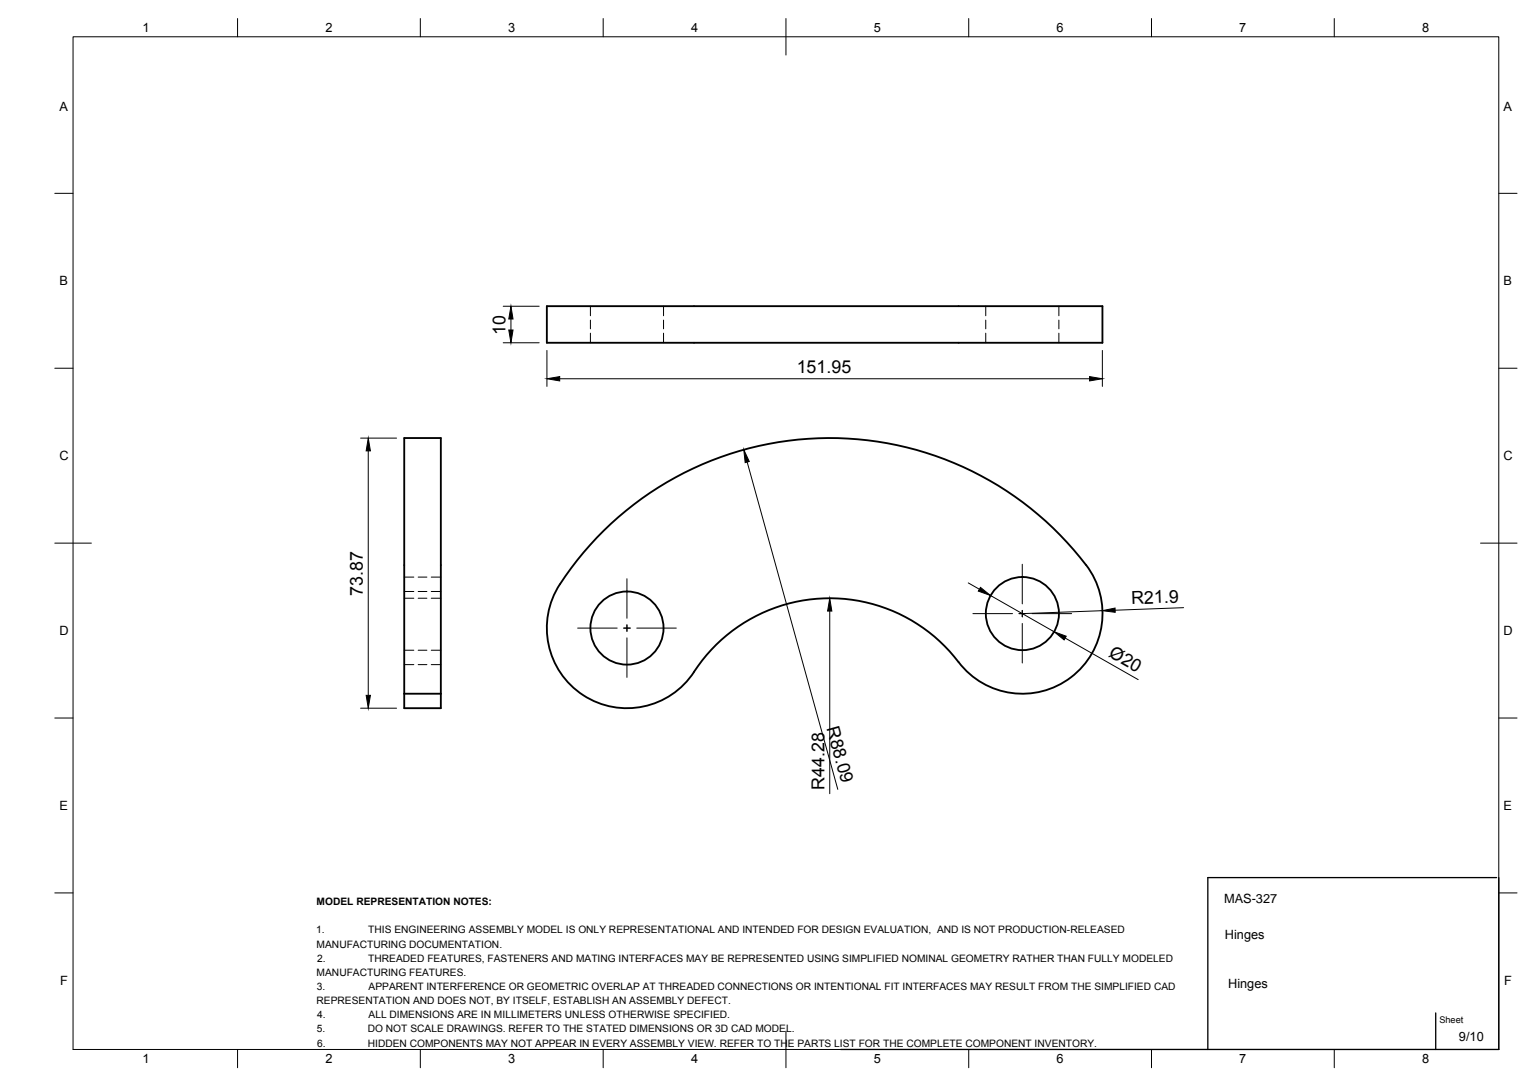
ISO-10303-21;
HEADER;
FILE_DESCRIPTION (('STEP AP214'),
    '1' );
FILE_NAME ('Hinges.step',
    '2026-10-06T22:16:42',
    ( '' ),
    ( '' ),
    'SwSTEP 2.0',
    'SolidWorks 2025',
    '' );
FILE_SCHEMA (( 'AUTOMOTIVE_DESIGN' ));
ENDSEC;

DATA;
#86=DIRECTION ( 'NONE',  ( 0.000000000000000000, 0.000000000000000000, 1.000000000000000000 ) ) ;
#206=AXIS2_PLACEMENT_3D ( 'NONE', #10122, #1740, #19817 ) ;
#240=DIRECTION ( 'NONE',  ( 0.000000000000000000, 0.000000000000000000, 1.000000000000000000 ) ) ;
#280=DIRECTION ( 'NONE',  ( -0.000000000000000000, -0.000000000000000000, -1.000000000000000000 ) ) ;
#386=DIRECTION ( 'NONE',  ( -1.000000000000000000, 0.000000000000000000, 0.000000000000000000 ) ) ;
#487=CARTESIAN_POINT ( 'NONE',  ( 147.5268905834513475, 193.0332408774651185, 14.00000000000001776 ) ) ;
#490=EDGE_CURVE ( 'NONE', #561, #602, #17397, .T. ) ;
#515=ORIENTED_EDGE ( 'NONE', *, *, #14295, .T. ) ;
#517=CARTESIAN_POINT ( 'NONE',  ( 159.4819454078502190, 211.3876867681337046, 14.00000000000001776 ) ) ;
#561=VERTEX_POINT ( 'NONE', #8931 ) ;
#598=CARTESIAN_POINT ( 'NONE',  ( 147.5268905834513475, 193.0332408774651185, 14.00000000000001776 ) ) ;
#602=VERTEX_POINT ( 'NONE', #3063 ) ;
#624=AXIS2_PLACEMENT_3D ( 'NONE', #1762, #13223, #18408 ) ;
#683=ORIENTED_EDGE ( 'NONE', *, *, #21000, .F. ) ;
#816=ORIENTED_EDGE ( 'NONE', *, *, #1747, .T. ) ;
#867=CYLINDRICAL_SURFACE ( 'NONE', #16262, 88.09373137032866907 ) ;
#906=CARTESIAN_POINT ( 'NONE',  ( 138.2149183826930425, 102.3264679885537305, 14.00000000000001776 ) ) ;
#911=CIRCLE ( 'NONE', #16036, 88.09373137032866907 ) ;
#917=CIRCLE ( 'NONE', #14285, 21.90454335994854063 ) ;
#947=CIRCLE ( 'NONE', #8357, 10.00000000000000888 ) ;
#963=SHAPE_REPRESENTATION_RELATIONSHIP ( 'NONE' , 'NONE' ,  #3970, #16628 ) ;
#966=ADVANCED_FACE ( 'NONE', ( #3402 ), #18495, .T. ) ;
#1001=EDGE_LOOP ( 'NONE', ( #7950, #11263, #15363, #5851 ) ) ;
#1043=FACE_OUTER_BOUND ( 'NONE', #2864, .T. ) ;
#1045=( LENGTH_UNIT ( ) NAMED_UNIT ( * ) SI_UNIT ( .MILLI., .METRE. ) );
#1216=ORIENTED_EDGE ( 'NONE', *, *, #20304, .F. ) ;
#1369=( NAMED_UNIT ( * ) PLANE_ANGLE_UNIT ( ) SI_UNIT ( $, .RADIAN. ) );
#1376=AXIS2_PLACEMENT_3D ( 'NONE', #4360, #21349, #17699 ) ;
#1501=PRODUCT ( 'Hinges', 'Hinges', '', ( #2695 ) ) ;
#1740=DIRECTION ( 'NONE',  ( 0.000000000000000000, 0.000000000000000000, 1.000000000000000000 ) ) ;
#1747=EDGE_CURVE ( 'NONE', #4207, #19742, #20682, .T. ) ;
#1762=CARTESIAN_POINT ( 'NONE',  ( 151.4773229304660731, 84.89323405393692212, 14.00000000000001776 ) ) ;
#1767=ORIENTED_EDGE ( 'NONE', *, *, #7862, .T. ) ;
#1776=( GEOMETRIC_REPRESENTATION_CONTEXT ( 3 ) GLOBAL_UNCERTAINTY_ASSIGNED_CONTEXT ( ( #14131 ) ) GLOBAL_UNIT_ASSIGNED_CONTEXT ( ( #2724, #2506, #19371 ) ) REPRESENTATION_CONTEXT ( 'NONE', 'WORKASPACE' ) );
#1809=CARTESIAN_POINT ( 'NONE',  ( 129.5727795705175822, 84.89323405393692212, 14.00000000000001776 ) ) ;
#1834=AXIS2_PLACEMENT_3D ( 'NONE', #598, #280, #19122 ) ;
#1849=CARTESIAN_POINT ( 'NONE',  ( 137.5268905834513191, 193.0332408774651185, 14.00000000000001776 ) ) ;
#1928=CARTESIAN_POINT ( 'NONE',  ( 129.5727795705175822, 84.89323405393692212, 4.000000000000021316 ) ) ;
#2018=EDGE_LOOP ( 'NONE', ( #1767, #3911, #17935, #2040 ) ) ;
#2040=ORIENTED_EDGE ( 'NONE', *, *, #6906, .T. ) ;
#2069=EDGE_CURVE ( 'NONE', #4207, #6019, #20285, .T. ) ;
#2144=CARTESIAN_POINT ( 'NONE',  ( 147.5268905834513475, 193.0332408774651185, 4.000000000000021316 ) ) ;
#2330=ORIENTED_EDGE ( 'NONE', *, *, #21000, .T. ) ;
#2368=CARTESIAN_POINT ( 'NONE',  ( 164.7397274782390184, 67.46000011932014218, 4.000000000000021316 ) ) ;
#2403=CARTESIAN_POINT ( 'NONE',  ( 0.000000000000000000, 0.000000000000000000, 0.000000000000000000 ) ) ;
#2440=ORIENTED_EDGE ( 'NONE', *, *, #14295, .F. ) ;
#2445=CARTESIAN_POINT ( 'NONE',  ( 135.5718357590524192, 174.6787949867965324, 4.000000000000021316 ) ) ;
#2506=( NAMED_UNIT ( * ) PLANE_ANGLE_UNIT ( ) SI_UNIT ( $, .RADIAN. ) );
#2688=CARTESIAN_POINT ( 'NONE',  ( 151.4773229304660731, 84.89323405393692212, 14.00000000000001776 ) ) ;
#2695=PRODUCT_CONTEXT ( 'NONE', #5614, 'mechanical' ) ;
#2724=( LENGTH_UNIT ( ) NAMED_UNIT ( * ) SI_UNIT ( .MILLI., .METRE. ) );
#2734=DIRECTION ( 'NONE',  ( -0.000000000000000000, -0.000000000000000000, -1.000000000000000000 ) ) ;
#2752=CARTESIAN_POINT ( 'NONE',  ( 151.4773229304660731, 84.89323405393692212, 14.00000000000001776 ) ) ;
#2786=AXIS2_PLACEMENT_3D ( 'NONE', #13218, #4841, #6619 ) ;
#2842=ORIENTED_EDGE ( 'NONE', *, *, #14486, .F. ) ;
#2864=EDGE_LOOP ( 'NONE', ( #515, #9206, #2842, #9559 ) ) ;
#2893=AXIS2_PLACEMENT_3D ( 'NONE', #7958, #11580, #15332 ) ;
#2901=VECTOR ( 'NONE', #20014, 1000.000000000000000 ) ;
#2935=LINE ( 'NONE', #21135, #17207 ) ;
#2946=DIRECTION ( 'NONE',  ( 1.000000000000000000, 0.000000000000000000, 0.000000000000000000 ) ) ;
#2953=ORIENTED_EDGE ( 'NONE', *, *, #7751, .T. ) ;
#3063=CARTESIAN_POINT ( 'NONE',  ( 141.4773229304660447, 84.89323405393692212, 4.000000000000021316 ) ) ;
#3069=CARTESIAN_POINT ( 'NONE',  ( 157.5268905834513475, 193.0332408774651185, 4.000000000000021316 ) ) ;
#3087=AXIS2_PLACEMENT_3D ( 'NONE', #5335, #10087, #8763 ) ;
#3283=CARTESIAN_POINT ( 'NONE',  ( 147.5268905834513475, 193.0332408774651185, 14.00000000000001776 ) ) ;
#3290=EDGE_CURVE ( 'NONE', #19742, #18253, #917, .T. ) ;
#3292=CARTESIAN_POINT ( 'NONE',  ( 138.2149183826930425, 102.3264679885537305, 4.000000000000021316 ) ) ;
#3361=UNCERTAINTY_MEASURE_WITH_UNIT (LENGTH_MEASURE( 1.000000000000000082E-05 ), #1045, 'distance_accuracy_value', 'NONE');
#3402=FACE_OUTER_BOUND ( 'NONE', #5526, .T. ) ;
#3453=CARTESIAN_POINT ( 'NONE',  ( 147.5268905834513475, 193.0332408774651185, 4.000000000000021316 ) ) ;
#3558=ORIENTED_EDGE ( 'NONE', *, *, #3290, .F. ) ;
#3605=FACE_BOUND ( 'NONE', #4278, .T. ) ;
#3678=ADVANCED_FACE ( 'NONE', ( #18042, #6479, #16173 ), #7816, .F. ) ;
#3802=CIRCLE ( 'NONE', #18591, 10.00000000000000888 ) ;
#3803=FACE_OUTER_BOUND ( 'NONE', #16547, .T. ) ;
#3855=EDGE_CURVE ( 'NONE', #8015, #10293, #8796, .T. ) ;
#3911=ORIENTED_EDGE ( 'NONE', *, *, #1747, .F. ) ;
#3934=DIRECTION ( 'NONE',  ( -0.000000000000000000, -0.000000000000000000, -1.000000000000000000 ) ) ;
#3947=EDGE_CURVE ( 'NONE', #16997, #8015, #3802, .T. ) ;
#3970=SHAPE_REPRESENTATION ( 'Hinges', ( #12657 ), #1776 ) ;
#3979=DIRECTION ( 'NONE',  ( 1.000000000000000000, 0.000000000000000000, 0.000000000000000000 ) ) ;
#4168=CARTESIAN_POINT ( 'NONE',  ( 151.4773229304660731, 84.89323405393692212, 4.000000000000021316 ) ) ;
#4173=EDGE_CURVE ( 'NONE', #18391, #12691, #19038, .T. ) ;
#4207=VERTEX_POINT ( 'NONE', #517 ) ;
#4278=EDGE_LOOP ( 'NONE', ( #15239, #11300 ) ) ;
#4339=CARTESIAN_POINT ( 'NONE',  ( 137.5268905834513191, 193.0332408774651185, 4.000000000000021316 ) ) ;
#4360=CARTESIAN_POINT ( 'NONE',  ( 147.5268905834513475, 193.0332408774651185, 14.00000000000001776 ) ) ;
#4487=FACE_OUTER_BOUND ( 'NONE', #2018, .T. ) ;
#4579=ORIENTED_EDGE ( 'NONE', *, *, #490, .T. ) ;
#4603=VERTEX_POINT ( 'NONE', #1928 ) ;
#4652=PRODUCT_DEFINITION_CONTEXT ( 'detailed design', #18727, 'design' ) ;
#4765=EDGE_LOOP ( 'NONE', ( #17772, #14554 ) ) ;
#4777=CARTESIAN_POINT ( 'NONE',  ( 164.7397274782390184, 67.46000011932014218, 14.00000000000001776 ) ) ;
#4841=DIRECTION ( 'NONE',  ( 0.000000000000000000, 0.000000000000000000, 1.000000000000000000 ) ) ;
#4901=EDGE_CURVE ( 'NONE', #13154, #4207, #12224, .T. ) ;
#4928=DIRECTION ( 'NONE',  ( 0.000000000000000000, 0.000000000000000000, 1.000000000000000000 ) ) ;
#4974=ORIENTED_EDGE ( 'NONE', *, *, #10822, .F. ) ;
#5039=FACE_OUTER_BOUND ( 'NONE', #10933, .T. ) ;
#5114=DIRECTION ( 'NONE',  ( -1.000000000000000000, 0.000000000000000000, 0.000000000000000000 ) ) ;
#5268=CIRCLE ( 'NONE', #6317, 10.00000000000000888 ) ;
#5335=CARTESIAN_POINT ( 'NONE',  ( 111.4021762516569964, 137.5714195593754710, 14.00000000000001776 ) ) ;
#5446=ORIENTED_EDGE ( 'NONE', *, *, #9283, .T. ) ;
#5526=EDGE_LOOP ( 'NONE', ( #7904, #7670, #21323, #21268 ) ) ;
#5567=CARTESIAN_POINT ( 'NONE',  ( 159.4819454078502190, 211.3876867681337046, 14.00000000000001776 ) ) ;
#5614=APPLICATION_CONTEXT ( 'automotive_design' ) ;
#5615=( GEOMETRIC_REPRESENTATION_CONTEXT ( 3 ) GLOBAL_UNCERTAINTY_ASSIGNED_CONTEXT ( ( #3361 ) ) GLOBAL_UNIT_ASSIGNED_CONTEXT ( ( #1045, #1369, #18113 ) ) REPRESENTATION_CONTEXT ( 'NONE', 'WORKASPACE' ) );
#5673=FACE_OUTER_BOUND ( 'NONE', #15781, .T. ) ;
#5779=CIRCLE ( 'NONE', #7222, 10.00000000000000888 ) ;
#5832=DIRECTION ( 'NONE',  ( -0.000000000000000000, -0.000000000000000000, -1.000000000000000000 ) ) ;
#5851=ORIENTED_EDGE ( 'NONE', *, *, #490, .F. ) ;
#5946=DIRECTION ( 'NONE',  ( -1.000000000000000000, 0.000000000000000000, 0.000000000000000000 ) ) ;
#6016=ORIENTED_EDGE ( 'NONE', *, *, #10822, .T. ) ;
#6019=VERTEX_POINT ( 'NONE', #21122 ) ;
#6046=PRODUCT_DEFINITION_SHAPE ( 'NONE', 'NONE',  #14706 ) ;
#6105=EDGE_CURVE ( 'NONE', #20206, #561, #8184, .T. ) ;
#6201=CARTESIAN_POINT ( 'NONE',  ( 147.5268905834513475, 193.0332408774651185, 4.000000000000021316 ) ) ;
#6257=VECTOR ( 'NONE', #7033, 1000.000000000000000 ) ;
#6296=CIRCLE ( 'NONE', #14048, 21.90454335994854063 ) ;
#6317=AXIS2_PLACEMENT_3D ( 'NONE', #2688, #17781, #7779 ) ;
#6329=SURFACE_SIDE_STYLE ('',( #14808 ) ) ;
#6365=CARTESIAN_POINT ( 'NONE',  ( 111.4021762516569964, 137.5714195593754710, 4.000000000000021316 ) ) ;
#6367=CARTESIAN_POINT ( 'NONE',  ( 131.4397495910615135, 111.2323268066561894, 4.000000000000021316 ) ) ;
#6390=ADVANCED_FACE ( 'NONE', ( #3605, #5039, #17031 ), #6811, .T. ) ;
#6439=CARTESIAN_POINT ( 'NONE',  ( 147.5268905834513475, 193.0332408774651185, 14.00000000000001776 ) ) ;
#6479=FACE_BOUND ( 'NONE', #21784, .T. ) ;
#6489=DIRECTION ( 'NONE',  ( 1.000000000000000000, 0.000000000000000000, 0.000000000000000000 ) ) ;
#6619=DIRECTION ( 'NONE',  ( 1.000000000000000000, 0.000000000000000000, 0.000000000000000000 ) ) ;
#6630=ORIENTED_EDGE ( 'NONE', *, *, #14584, .F. ) ;
#6719=DIRECTION ( 'NONE',  ( -1.000000000000000000, 0.000000000000000000, 0.000000000000000000 ) ) ;
#6811=PLANE ( 'NONE',  #18735 ) ;
#6883=CYLINDRICAL_SURFACE ( 'NONE', #18176, 21.90454335994848734 ) ;
#6900=CYLINDRICAL_SURFACE ( 'NONE', #19935, 21.90454335994854063 ) ;
#6906=EDGE_CURVE ( 'NONE', #13154, #10374, #20438, .T. ) ;
#6958=AXIS2_PLACEMENT_3D ( 'NONE', #7777, #21221, #9647 ) ;
#7033=DIRECTION ( 'NONE',  ( -0.000000000000000000, -0.000000000000000000, -1.000000000000000000 ) ) ;
#7050=DIRECTION ( 'NONE',  ( 0.000000000000000000, 0.000000000000000000, 1.000000000000000000 ) ) ;
#7108=CARTESIAN_POINT ( 'NONE',  ( 147.5268905834513475, 193.0332408774651185, 14.00000000000001776 ) ) ;
#7162=CARTESIAN_POINT ( 'NONE',  ( 147.5268905834513475, 193.0332408774651185, 14.00000000000001776 ) ) ;
#7222=AXIS2_PLACEMENT_3D ( 'NONE', #4168, #9140, #10897 ) ;
#7225=DIRECTION ( 'NONE',  ( -0.000000000000000000, -0.000000000000000000, -1.000000000000000000 ) ) ;
#7363=EDGE_CURVE ( 'NONE', #13378, #13154, #7385, .T. ) ;
#7369=CIRCLE ( 'NONE', #1376, 10.00000000000000888 ) ;
#7385=CIRCLE ( 'NONE', #2786, 21.90454335994848734 ) ;
#7398=COLOUR_RGB ( '', 0.09019608, 0.27058824, 0.51372549) ;
#7494=EDGE_CURVE ( 'NONE', #20206, #19334, #17273, .T. ) ;
#7511=LINE ( 'NONE', #14210, #17134 ) ;
#7616=AXIS2_PLACEMENT_3D ( 'NONE', #2144, #8877, #15584 ) ;
#7622=CYLINDRICAL_SURFACE ( 'NONE', #7907, 10.00000000000000888 ) ;
#7670=ORIENTED_EDGE ( 'NONE', *, *, #9283, .F. ) ;
#7682=SHAPE_DEFINITION_REPRESENTATION ( #6046, #3970 ) ;
#7750=ORIENTED_EDGE ( 'NONE', *, *, #6906, .F. ) ;
#7751=EDGE_CURVE ( 'NONE', #13378, #4603, #16490, .T. ) ;
#7772=ORIENTED_EDGE ( 'NONE', *, *, #20824, .T. ) ;
#7777=CARTESIAN_POINT ( 'NONE',  ( 111.4021762516569964, 137.5714195593754710, 14.00000000000001776 ) ) ;
#7779=DIRECTION ( 'NONE',  ( 1.000000000000000000, 0.000000000000000000, 0.000000000000000000 ) ) ;
#7816=PLANE ( 'NONE',  #10148 ) ;
#7862=EDGE_CURVE ( 'NONE', #10374, #19742, #911, .T. ) ;
#7877=EDGE_CURVE ( 'NONE', #20239, #10293, #9724, .T. ) ;
#7891=EDGE_CURVE ( 'NONE', #4603, #10374, #15355, .T. ) ;
#7904=ORIENTED_EDGE ( 'NONE', *, *, #7751, .F. ) ;
#7907=AXIS2_PLACEMENT_3D ( 'NONE', #12782, #15866, #5946 ) ;
#7950=ORIENTED_EDGE ( 'NONE', *, *, #21656, .T. ) ;
#7957=ORIENTED_EDGE ( 'NONE', *, *, #2069, .T. ) ;
#7958=CARTESIAN_POINT ( 'NONE',  ( 151.4773229304660731, 84.89323405393692212, 4.000000000000021316 ) ) ;
#7988=ORIENTED_EDGE ( 'NONE', *, *, #14486, .T. ) ;
#8015=VERTEX_POINT ( 'NONE', #12411 ) ;
#8184=CIRCLE ( 'NONE', #8539, 10.00000000000000888 ) ;
#8322=CARTESIAN_POINT ( 'NONE',  ( 164.7397274782390184, 67.46000011932014218, 14.00000000000001776 ) ) ;
#8339=DIRECTION ( 'NONE',  ( -0.000000000000000000, -0.000000000000000000, -1.000000000000000000 ) ) ;
#8357=AXIS2_PLACEMENT_3D ( 'NONE', #12124, #15762, #3979 ) ;
#8363=CARTESIAN_POINT ( 'NONE',  ( 151.4773229304660731, 84.89323405393692212, 14.00000000000001776 ) ) ;
#8422=CARTESIAN_POINT ( 'NONE',  ( 157.5268905834513475, 193.0332408774651185, 14.00000000000001776 ) ) ;
#8474=CARTESIAN_POINT ( 'NONE',  ( 129.5727795705175822, 84.89323405393692212, 14.00000000000001776 ) ) ;
#8475=CLOSED_SHELL ( 'NONE', ( #9761, #18925, #8585, #13380, #6390, #3678, #966, #17842, #16477, #10699, #12632, #10454 ) ) ;
#8539=AXIS2_PLACEMENT_3D ( 'NONE', #11096, #13079, #17808 ) ;
#8565=EDGE_CURVE ( 'NONE', #18253, #13487, #18870, .T. ) ;
#8585=ADVANCED_FACE ( 'NONE', ( #3803 ), #6900, .T. ) ;
#8596=FACE_OUTER_BOUND ( 'NONE', #20913, .T. ) ;
#8763=DIRECTION ( 'NONE',  ( 1.000000000000000000, 0.000000000000000000, 0.000000000000000000 ) ) ;
#8773=CYLINDRICAL_SURFACE ( 'NONE', #1834, 21.90454335994854063 ) ;
#8796=LINE ( 'NONE', #1849, #6257 ) ;
#8877=DIRECTION ( 'NONE',  ( 0.000000000000000000, 0.000000000000000000, 1.000000000000000000 ) ) ;
#8931=CARTESIAN_POINT ( 'NONE',  ( 141.4773229304660447, 84.89323405393692212, 14.00000000000001776 ) ) ;
#8933=EDGE_LOOP ( 'NONE', ( #11196, #15122, #816, #15559 ) ) ;
#8990=DIRECTION ( 'NONE',  ( -0.000000000000000000, -0.000000000000000000, -1.000000000000000000 ) ) ;
#9103=EDGE_LOOP ( 'NONE', ( #19441, #11957, #4579, #4974 ) ) ;
#9140=DIRECTION ( 'NONE',  ( 0.000000000000000000, 0.000000000000000000, 1.000000000000000000 ) ) ;
#9206=ORIENTED_EDGE ( 'NONE', *, *, #4173, .F. ) ;
#9283=EDGE_CURVE ( 'NONE', #18391, #13378, #20702, .T. ) ;
#9312=DIRECTION ( 'NONE',  ( 1.000000000000000000, 0.000000000000000000, 0.000000000000000000 ) ) ;
#9368=VECTOR ( 'NONE', #14738, 1000.000000000000000 ) ;
#9396=CIRCLE ( 'NONE', #12198, 44.28464465043163756 ) ;
#9422=DIRECTION ( 'NONE',  ( 1.000000000000000000, 0.000000000000000000, 0.000000000000000000 ) ) ;
#9492=FACE_OUTER_BOUND ( 'NONE', #1001, .T. ) ;
#9559=ORIENTED_EDGE ( 'NONE', *, *, #14093, .T. ) ;
#9647=DIRECTION ( 'NONE',  ( -1.000000000000000000, 0.000000000000000000, 0.000000000000000000 ) ) ;
#9687=CARTESIAN_POINT ( 'NONE',  ( 151.4773229304660731, 84.89323405393692212, 4.000000000000021316 ) ) ;
#9697=CARTESIAN_POINT ( 'NONE',  ( 161.4773229304660731, 84.89323405393692212, 14.00000000000001776 ) ) ;
#9724=CIRCLE ( 'NONE', #206, 10.00000000000000888 ) ;
#9761=ADVANCED_FACE ( 'NONE', ( #8596 ), #20280, .F. ) ;
#9995=CARTESIAN_POINT ( 'NONE',  ( 135.5718357590524192, 174.6787949867965324, 14.00000000000001776 ) ) ;
#10087=DIRECTION ( 'NONE',  ( 0.000000000000000000, 0.000000000000000000, 1.000000000000000000 ) ) ;
#10122=CARTESIAN_POINT ( 'NONE',  ( 147.5268905834513475, 193.0332408774651185, 4.000000000000021316 ) ) ;
#10148=AXIS2_PLACEMENT_3D ( 'NONE', #6367, #14521, #21261 ) ;
#10218=PRODUCT_DEFINITION_FORMATION_WITH_SPECIFIED_SOURCE ( 'ANY', '', #1501, .NOT_KNOWN. ) ;
#10286=ORIENTED_EDGE ( 'NONE', *, *, #7877, .F. ) ;
#10293=VERTEX_POINT ( 'NONE', #4339 ) ;
#10374=VERTEX_POINT ( 'NONE', #2368 ) ;
#10454=ADVANCED_FACE ( 'NONE', ( #5673 ), #19130, .F. ) ;
#10536=ORIENTED_EDGE ( 'NONE', *, *, #15749, .F. ) ;
#10561=STYLED_ITEM ( 'NONE', ( #13055 ), #21708 ) ;
#10584=DIRECTION ( 'NONE',  ( -0.000000000000000000, -0.000000000000000000, -1.000000000000000000 ) ) ;
#10640=FACE_OUTER_BOUND ( 'NONE', #8933, .T. ) ;
#10680=DIRECTION ( 'NONE',  ( -1.000000000000000000, 0.000000000000000000, 0.000000000000000000 ) ) ;
#10699=ADVANCED_FACE ( 'NONE', ( #1043 ), #14699, .F. ) ;
#10822=EDGE_CURVE ( 'NONE', #19334, #602, #947, .T. ) ;
#10862=CARTESIAN_POINT ( 'NONE',  ( 111.4021762516569964, 137.5714195593754710, 4.000000000000021316 ) ) ;
#10897=DIRECTION ( 'NONE',  ( 1.000000000000000000, 0.000000000000000000, 0.000000000000000000 ) ) ;
#10933=EDGE_LOOP ( 'NONE', ( #5446, #16391, #17909, #7957, #18415, #7988 ) ) ;
#11096=CARTESIAN_POINT ( 'NONE',  ( 151.4773229304660731, 84.89323405393692212, 14.00000000000001776 ) ) ;
#11109=CARTESIAN_POINT ( 'NONE',  ( 111.4021762516569964, 137.5714195593754710, 14.00000000000001776 ) ) ;
#11196=ORIENTED_EDGE ( 'NONE', *, *, #20824, .F. ) ;
#11217=ORIENTED_EDGE ( 'NONE', *, *, #14093, .F. ) ;
#11233=EDGE_CURVE ( 'NONE', #16997, #20239, #7511, .T. ) ;
#11263=ORIENTED_EDGE ( 'NONE', *, *, #7494, .T. ) ;
#11283=FILL_AREA_STYLE_COLOUR ( '', #7398 ) ;
#11300=ORIENTED_EDGE ( 'NONE', *, *, #6105, .F. ) ;
#11310=CARTESIAN_POINT ( 'NONE',  ( 159.4819454078502190, 211.3876867681337046, 4.000000000000021316 ) ) ;
#11501=DIRECTION ( 'NONE',  ( -1.000000000000000000, 0.000000000000000000, 0.000000000000000000 ) ) ;
#11580=DIRECTION ( 'NONE',  ( 0.000000000000000000, 0.000000000000000000, 1.000000000000000000 ) ) ;
#11639=DIRECTION ( 'NONE',  ( 1.000000000000000000, 0.000000000000000000, -0.000000000000000000 ) ) ;
#11780=CARTESIAN_POINT ( 'NONE',  ( 161.4773229304660731, 84.89323405393692212, 14.00000000000001776 ) ) ;
#11856=AXIS2_PLACEMENT_3D ( 'NONE', #7162, #17275, #10680 ) ;
#11859=CIRCLE ( 'NONE', #19959, 44.28464465043163756 ) ;
#11957=ORIENTED_EDGE ( 'NONE', *, *, #6105, .T. ) ;
#11970=CARTESIAN_POINT ( 'NONE',  ( 131.4397495910615135, 111.2323268066561894, 14.00000000000001776 ) ) ;
#12124=CARTESIAN_POINT ( 'NONE',  ( 151.4773229304660731, 84.89323405393692212, 4.000000000000021316 ) ) ;
#12194=AXIS2_PLACEMENT_3D ( 'NONE', #2752, #12676, #21280 ) ;
#12198=AXIS2_PLACEMENT_3D ( 'NONE', #10862, #8990, #9312 ) ;
#12224=CIRCLE ( 'NONE', #3087, 88.09373137032866907 ) ;
#12289=DIRECTION ( 'NONE',  ( -0.000000000000000000, -0.000000000000000000, -1.000000000000000000 ) ) ;
#12411=CARTESIAN_POINT ( 'NONE',  ( 137.5268905834513191, 193.0332408774651185, 14.00000000000001776 ) ) ;
#12528=AXIS2_PLACEMENT_3D ( 'NONE', #9687, #18490, #21806 ) ;
#12552=CARTESIAN_POINT ( 'NONE',  ( 141.4773229304660447, 84.89323405393692212, 14.00000000000001776 ) ) ;
#12632=ADVANCED_FACE ( 'NONE', ( #15317 ), #21720, .F. ) ;
#12657=AXIS2_PLACEMENT_3D ( 'NONE', #2403, #7050, #17169 ) ;
#12676=DIRECTION ( 'NONE',  ( 0.000000000000000000, 0.000000000000000000, 1.000000000000000000 ) ) ;
#12691=VERTEX_POINT ( 'NONE', #3292 ) ;
#12782=CARTESIAN_POINT ( 'NONE',  ( 151.4773229304660731, 84.89323405393692212, 14.00000000000001776 ) ) ;
#12802=ORIENTED_EDGE ( 'NONE', *, *, #19592, .T. ) ;
#12986=DIRECTION ( 'NONE',  ( -1.000000000000000000, 0.000000000000000000, 0.000000000000000000 ) ) ;
#13055=PRESENTATION_STYLE_ASSIGNMENT (( #19448 ) ) ;
#13079=DIRECTION ( 'NONE',  ( 0.000000000000000000, 0.000000000000000000, 1.000000000000000000 ) ) ;
#13154=VERTEX_POINT ( 'NONE', #4777 ) ;
#13218=CARTESIAN_POINT ( 'NONE',  ( 151.4773229304660731, 84.89323405393692212, 14.00000000000001776 ) ) ;
#13223=DIRECTION ( 'NONE',  ( -0.000000000000000000, -0.000000000000000000, -1.000000000000000000 ) ) ;
#13378=VERTEX_POINT ( 'NONE', #1809 ) ;
#13380=ADVANCED_FACE ( 'NONE', ( #17000 ), #6883, .T. ) ;
#13480=ORIENTED_EDGE ( 'NONE', *, *, #7891, .F. ) ;
#13487=VERTEX_POINT ( 'NONE', #2445 ) ;
#13489=DIRECTION ( 'NONE',  ( -0.000000000000000000, -0.000000000000000000, -1.000000000000000000 ) ) ;
#13527=DIRECTION ( 'NONE',  ( 1.000000000000000000, 0.000000000000000000, 0.000000000000000000 ) ) ;
#13813=DIRECTION ( 'NONE',  ( 0.000000000000000000, 0.000000000000000000, 1.000000000000000000 ) ) ;
#13910=VECTOR ( 'NONE', #12289, 1000.000000000000000 ) ;
#13941=VECTOR ( 'NONE', #8339, 1000.000000000000000 ) ;
#13995=VECTOR ( 'NONE', #3934, 1000.000000000000000 ) ;
#14048=AXIS2_PLACEMENT_3D ( 'NONE', #14748, #18162, #6489 ) ;
#14093=EDGE_CURVE ( 'NONE', #14386, #13487, #20136, .T. ) ;
#14131=UNCERTAINTY_MEASURE_WITH_UNIT (LENGTH_MEASURE( 1.000000000000000082E-05 ), #2724, 'distance_accuracy_value', 'NONE');
#14178=EDGE_LOOP ( 'NONE', ( #6630, #2440, #16753, #3558, #17616, #13480 ) ) ;
#14210=CARTESIAN_POINT ( 'NONE',  ( 157.5268905834513475, 193.0332408774651185, 14.00000000000001776 ) ) ;
#14285=AXIS2_PLACEMENT_3D ( 'NONE', #6201, #17988, #21102 ) ;
#14295=EDGE_CURVE ( 'NONE', #13487, #12691, #9396, .T. ) ;
#14386=VERTEX_POINT ( 'NONE', #21657 ) ;
#14413=MECHANICAL_DESIGN_GEOMETRIC_PRESENTATION_REPRESENTATION('',(#10561),#5615);
#14486=EDGE_CURVE ( 'NONE', #14386, #18391, #11859, .T. ) ;
#14521=DIRECTION ( 'NONE',  ( 0.000000000000000000, 0.000000000000000000, 1.000000000000000000 ) ) ;
#14554=ORIENTED_EDGE ( 'NONE', *, *, #7877, .T. ) ;
#14556=ORIENTED_EDGE ( 'NONE', *, *, #3947, .F. ) ;
#14584=EDGE_CURVE ( 'NONE', #12691, #4603, #18744, .T. ) ;
#14692=DIRECTION ( 'NONE',  ( -0.000000000000000000, -0.000000000000000000, -1.000000000000000000 ) ) ;
#14699=CYLINDRICAL_SURFACE ( 'NONE', #6958, 44.28464465043163756 ) ;
#14706=PRODUCT_DEFINITION ( 'UNKNOWN', '', #10218, #4652 ) ;
#14725=DIRECTION ( 'NONE',  ( -0.000000000000000000, -0.000000000000000000, -1.000000000000000000 ) ) ;
#14738=DIRECTION ( 'NONE',  ( -0.000000000000000000, -0.000000000000000000, -1.000000000000000000 ) ) ;
#14748=CARTESIAN_POINT ( 'NONE',  ( 147.5268905834513475, 193.0332408774651185, 14.00000000000001776 ) ) ;
#14808=SURFACE_STYLE_FILL_AREA ( #21438 ) ;
#15029=AXIS2_PLACEMENT_3D ( 'NONE', #6439, #16349, #11501 ) ;
#15122=ORIENTED_EDGE ( 'NONE', *, *, #2069, .F. ) ;
#15203=CIRCLE ( 'NONE', #16239, 10.00000000000000888 ) ;
#15239=ORIENTED_EDGE ( 'NONE', *, *, #21656, .F. ) ;
#15317=FACE_OUTER_BOUND ( 'NONE', #9103, .T. ) ;
#15332=DIRECTION ( 'NONE',  ( 1.000000000000000000, 0.000000000000000000, 0.000000000000000000 ) ) ;
#15355=CIRCLE ( 'NONE', #12528, 21.90454335994848734 ) ;
#15363=ORIENTED_EDGE ( 'NONE', *, *, #19592, .F. ) ;
#15559=ORIENTED_EDGE ( 'NONE', *, *, #3290, .T. ) ;
#15584=DIRECTION ( 'NONE',  ( 1.000000000000000000, 0.000000000000000000, 0.000000000000000000 ) ) ;
#15749=EDGE_CURVE ( 'NONE', #10293, #20239, #15203, .T. ) ;
#15762=DIRECTION ( 'NONE',  ( 0.000000000000000000, 0.000000000000000000, 1.000000000000000000 ) ) ;
#15781=EDGE_LOOP ( 'NONE', ( #19602, #16772, #21372, #10286 ) ) ;
#15866=DIRECTION ( 'NONE',  ( -0.000000000000000000, -0.000000000000000000, -1.000000000000000000 ) ) ;
#16036=AXIS2_PLACEMENT_3D ( 'NONE', #6365, #19931, #2946 ) ;
#16173=FACE_BOUND ( 'NONE', #4765, .T. ) ;
#16239=AXIS2_PLACEMENT_3D ( 'NONE', #3453, #240, #17092 ) ;
#16262=AXIS2_PLACEMENT_3D ( 'NONE', #11109, #2734, #12986 ) ;
#16349=DIRECTION ( 'NONE',  ( -0.000000000000000000, -0.000000000000000000, -1.000000000000000000 ) ) ;
#16391=ORIENTED_EDGE ( 'NONE', *, *, #7363, .T. ) ;
#16469=ORIENTED_EDGE ( 'NONE', *, *, #3855, .F. ) ;
#16477=ADVANCED_FACE ( 'NONE', ( #10640 ), #8773, .T. ) ;
#16490=LINE ( 'NONE', #8474, #9368 ) ;
#16547=EDGE_LOOP ( 'NONE', ( #1216, #7772, #20967, #11217 ) ) ;
#16628=ADVANCED_BREP_SHAPE_REPRESENTATION ( '', ( #21708, #12657 ), #1776 ) ;
#16676=CARTESIAN_POINT ( 'NONE',  ( 151.4773229304660731, 84.89323405393692212, 14.00000000000001776 ) ) ;
#16753=ORIENTED_EDGE ( 'NONE', *, *, #8565, .F. ) ;
#16772=ORIENTED_EDGE ( 'NONE', *, *, #3947, .T. ) ;
#16997=VERTEX_POINT ( 'NONE', #8422 ) ;
#17000=FACE_OUTER_BOUND ( 'NONE', #18848, .T. ) ;
#17031=FACE_BOUND ( 'NONE', #20941, .T. ) ;
#17092=DIRECTION ( 'NONE',  ( 1.000000000000000000, 0.000000000000000000, 0.000000000000000000 ) ) ;
#17134=VECTOR ( 'NONE', #5832, 1000.000000000000000 ) ;
#17169=DIRECTION ( 'NONE',  ( 1.000000000000000000, 0.000000000000000000, 0.000000000000000000 ) ) ;
#17207=VECTOR ( 'NONE', #14725, 1000.000000000000000 ) ;
#17257=CARTESIAN_POINT ( 'NONE',  ( 138.2149183826930425, 102.3264679885537305, 14.00000000000001776 ) ) ;
#17273=LINE ( 'NONE', #11780, #17739 ) ;
#17275=DIRECTION ( 'NONE',  ( -0.000000000000000000, -0.000000000000000000, -1.000000000000000000 ) ) ;
#17397=LINE ( 'NONE', #12552, #18693 ) ;
#17434=CARTESIAN_POINT ( 'NONE',  ( 125.6223472235027998, 193.0332408774651185, 4.000000000000021316 ) ) ;
#17616=ORIENTED_EDGE ( 'NONE', *, *, #7862, .F. ) ;
#17699=DIRECTION ( 'NONE',  ( 1.000000000000000000, 0.000000000000000000, 0.000000000000000000 ) ) ;
#17707=CARTESIAN_POINT ( 'NONE',  ( 161.4773229304660731, 84.89323405393692212, 4.000000000000021316 ) ) ;
#17739=VECTOR ( 'NONE', #18509, 1000.000000000000000 ) ;
#17772=ORIENTED_EDGE ( 'NONE', *, *, #15749, .T. ) ;
#17781=DIRECTION ( 'NONE',  ( 0.000000000000000000, 0.000000000000000000, 1.000000000000000000 ) ) ;
#17808=DIRECTION ( 'NONE',  ( 1.000000000000000000, 0.000000000000000000, 0.000000000000000000 ) ) ;
#17842=ADVANCED_FACE ( 'NONE', ( #4487 ), #867, .T. ) ;
#17909=ORIENTED_EDGE ( 'NONE', *, *, #4901, .T. ) ;
#17935=ORIENTED_EDGE ( 'NONE', *, *, #4901, .F. ) ;
#17988=DIRECTION ( 'NONE',  ( 0.000000000000000000, 0.000000000000000000, 1.000000000000000000 ) ) ;
#18042=FACE_OUTER_BOUND ( 'NONE', #14178, .T. ) ;
#18077=ORIENTED_EDGE ( 'NONE', *, *, #7363, .F. ) ;
#18113=( NAMED_UNIT ( * ) SI_UNIT ( $, .STERADIAN. ) SOLID_ANGLE_UNIT ( ) );
#18162=DIRECTION ( 'NONE',  ( 0.000000000000000000, 0.000000000000000000, 1.000000000000000000 ) ) ;
#18176=AXIS2_PLACEMENT_3D ( 'NONE', #16676, #13489, #5114 ) ;
#18223=CARTESIAN_POINT ( 'NONE',  ( 111.4021762516569964, 137.5714195593754710, 14.00000000000001776 ) ) ;
#18253=VERTEX_POINT ( 'NONE', #17434 ) ;
#18391=VERTEX_POINT ( 'NONE', #906 ) ;
#18408=DIRECTION ( 'NONE',  ( -1.000000000000000000, 0.000000000000000000, 0.000000000000000000 ) ) ;
#18415=ORIENTED_EDGE ( 'NONE', *, *, #20304, .T. ) ;
#18490=DIRECTION ( 'NONE',  ( 0.000000000000000000, 0.000000000000000000, 1.000000000000000000 ) ) ;
#18495=CYLINDRICAL_SURFACE ( 'NONE', #20268, 21.90454335994848734 ) ;
#18509=DIRECTION ( 'NONE',  ( -0.000000000000000000, -0.000000000000000000, -1.000000000000000000 ) ) ;
#18591=AXIS2_PLACEMENT_3D ( 'NONE', #3283, #86, #13527 ) ;
#18693=VECTOR ( 'NONE', #10584, 1000.000000000000000 ) ;
#18727=APPLICATION_CONTEXT ( 'automotive_design' ) ;
#18735=AXIS2_PLACEMENT_3D ( 'NONE', #11970, #4928, #11639 ) ;
#18744=CIRCLE ( 'NONE', #2893, 21.90454335994848734 ) ;
#18848=EDGE_LOOP ( 'NONE', ( #18077, #2953, #18868, #7750 ) ) ;
#18858=AXIS2_PLACEMENT_3D ( 'NONE', #7108, #13813, #20337 ) ;
#18868=ORIENTED_EDGE ( 'NONE', *, *, #7891, .T. ) ;
#18870=CIRCLE ( 'NONE', #7616, 21.90454335994854063 ) ;
#18925=ADVANCED_FACE ( 'NONE', ( #9492 ), #7622, .F. ) ;
#19038=LINE ( 'NONE', #17257, #13995 ) ;
#19122=DIRECTION ( 'NONE',  ( -1.000000000000000000, 0.000000000000000000, 0.000000000000000000 ) ) ;
#19130=CYLINDRICAL_SURFACE ( 'NONE', #15029, 10.00000000000000888 ) ;
#19334=VERTEX_POINT ( 'NONE', #17707 ) ;
#19371=( NAMED_UNIT ( * ) SI_UNIT ( $, .STERADIAN. ) SOLID_ANGLE_UNIT ( ) );
#19441=ORIENTED_EDGE ( 'NONE', *, *, #7494, .F. ) ;
#19448=SURFACE_STYLE_USAGE ( .BOTH. , #6329 ) ;
#19592=EDGE_CURVE ( 'NONE', #602, #19334, #5779, .T. ) ;
#19602=ORIENTED_EDGE ( 'NONE', *, *, #11233, .F. ) ;
#19742=VERTEX_POINT ( 'NONE', #11310 ) ;
#19817=DIRECTION ( 'NONE',  ( 1.000000000000000000, 0.000000000000000000, 0.000000000000000000 ) ) ;
#19931=DIRECTION ( 'NONE',  ( 0.000000000000000000, 0.000000000000000000, 1.000000000000000000 ) ) ;
#19935=AXIS2_PLACEMENT_3D ( 'NONE', #487, #7225, #386 ) ;
#19959=AXIS2_PLACEMENT_3D ( 'NONE', #18223, #14692, #9422 ) ;
#20014=DIRECTION ( 'NONE',  ( -0.000000000000000000, -0.000000000000000000, -1.000000000000000000 ) ) ;
#20136=LINE ( 'NONE', #9995, #13941 ) ;
#20206=VERTEX_POINT ( 'NONE', #9697 ) ;
#20239=VERTEX_POINT ( 'NONE', #3069 ) ;
#20268=AXIS2_PLACEMENT_3D ( 'NONE', #8363, #21810, #6719 ) ;
#20280=CYLINDRICAL_SURFACE ( 'NONE', #11856, 10.00000000000000888 ) ;
#20285=CIRCLE ( 'NONE', #18858, 21.90454335994854063 ) ;
#20304=EDGE_CURVE ( 'NONE', #6019, #14386, #6296, .T. ) ;
#20337=DIRECTION ( 'NONE',  ( 1.000000000000000000, 0.000000000000000000, 0.000000000000000000 ) ) ;
#20438=LINE ( 'NONE', #8322, #2901 ) ;
#20682=LINE ( 'NONE', #5567, #13910 ) ;
#20702=CIRCLE ( 'NONE', #12194, 21.90454335994848734 ) ;
#20824=EDGE_CURVE ( 'NONE', #6019, #18253, #2935, .T. ) ;
#20886=ORIENTED_EDGE ( 'NONE', *, *, #11233, .T. ) ;
#20913=EDGE_LOOP ( 'NONE', ( #2330, #20886, #10536, #16469 ) ) ;
#20941=EDGE_LOOP ( 'NONE', ( #683, #14556 ) ) ;
#20967=ORIENTED_EDGE ( 'NONE', *, *, #8565, .T. ) ;
#21000=EDGE_CURVE ( 'NONE', #8015, #16997, #7369, .T. ) ;
#21102=DIRECTION ( 'NONE',  ( 1.000000000000000000, 0.000000000000000000, 0.000000000000000000 ) ) ;
#21122=CARTESIAN_POINT ( 'NONE',  ( 125.6223472235027998, 193.0332408774651185, 14.00000000000001776 ) ) ;
#21135=CARTESIAN_POINT ( 'NONE',  ( 125.6223472235027998, 193.0332408774651185, 14.00000000000001776 ) ) ;
#21221=DIRECTION ( 'NONE',  ( -0.000000000000000000, -0.000000000000000000, -1.000000000000000000 ) ) ;
#21261=DIRECTION ( 'NONE',  ( 1.000000000000000000, 0.000000000000000000, -0.000000000000000000 ) ) ;
#21268=ORIENTED_EDGE ( 'NONE', *, *, #14584, .T. ) ;
#21280=DIRECTION ( 'NONE',  ( 1.000000000000000000, 0.000000000000000000, 0.000000000000000000 ) ) ;
#21323=ORIENTED_EDGE ( 'NONE', *, *, #4173, .T. ) ;
#21349=DIRECTION ( 'NONE',  ( 0.000000000000000000, 0.000000000000000000, 1.000000000000000000 ) ) ;
#21372=ORIENTED_EDGE ( 'NONE', *, *, #3855, .T. ) ;
#21438=FILL_AREA_STYLE ('',( #11283 ) ) ;
#21656=EDGE_CURVE ( 'NONE', #561, #20206, #5268, .T. ) ;
#21657=CARTESIAN_POINT ( 'NONE',  ( 135.5718357590524192, 174.6787949867965324, 14.00000000000001776 ) ) ;
#21708=MANIFOLD_SOLID_BREP ( 'Boss-Extrude7', #8475 ) ;
#21720=CYLINDRICAL_SURFACE ( 'NONE', #624, 10.00000000000000888 ) ;
#21784=EDGE_LOOP ( 'NONE', ( #12802, #6016 ) ) ;
#21806=DIRECTION ( 'NONE',  ( 1.000000000000000000, 0.000000000000000000, 0.000000000000000000 ) ) ;
#21810=DIRECTION ( 'NONE',  ( -0.000000000000000000, -0.000000000000000000, -1.000000000000000000 ) ) ;
ENDSEC;
END-ISO-10303-21;
